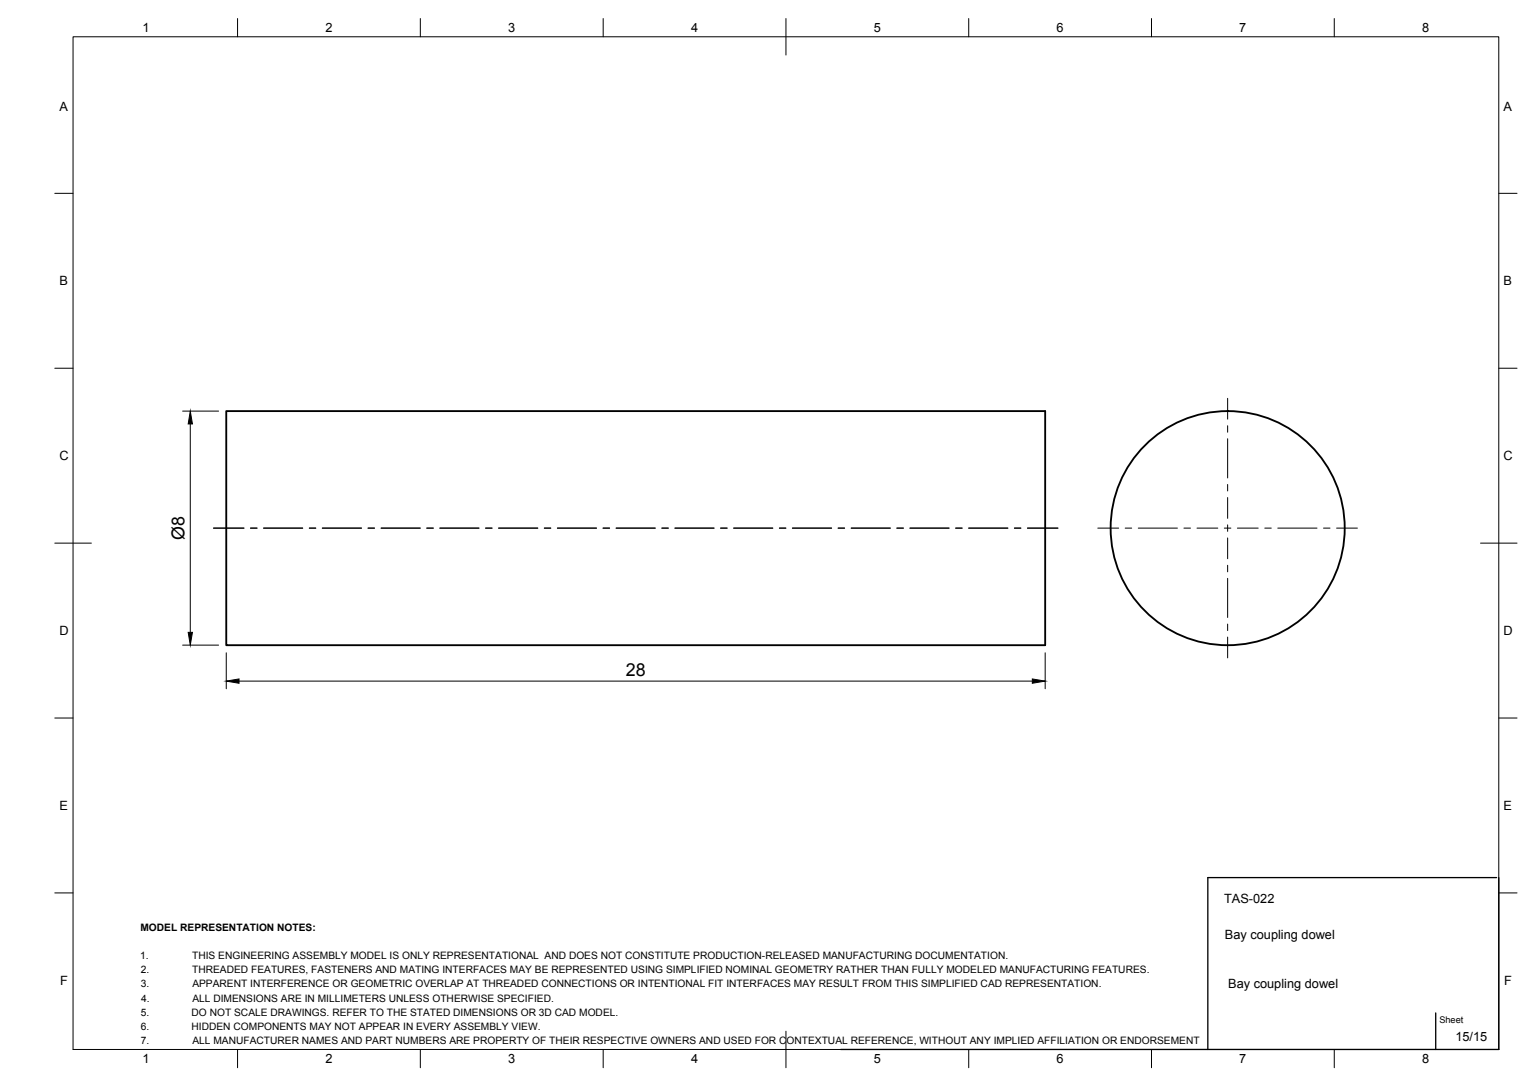
ISO-10303-21;
HEADER;
/* Generated by software containing ST-Developer
 * from STEP Tools, Inc. (www.steptools.com) 
 */

FILE_DESCRIPTION(
/* description */ (''),
/* implementation_level */ '2;1');

FILE_NAME(
/* name */ 'Bay coupling dowel.step',
/* time_stamp */ '2026-11-15T21:02:08-08:00',
/* author */ (''),
/* organization */ (''),
/* preprocessor_version */ 'ST-DEVELOPER v20.2',
/* originating_system */ 'Autodesk Translation Framework v15.17.0.0',
/* authorisation */ '');

FILE_SCHEMA (('AUTOMOTIVE_DESIGN { 1 0 10303 214 3 1 1 }'));
ENDSEC;

DATA;
#10=MECHANICAL_DESIGN_GEOMETRIC_PRESENTATION_REPRESENTATION('',(#616),#31566);
#488=CIRCLE('',#6246,0.4);
#489=CIRCLE('',#6247,0.4);
#571=CYLINDRICAL_SURFACE('',#6245,0.4);
#586=SHAPE_REPRESENTATION_RELATIONSHIP('SRR','None',#31650,#601);
#601=ADVANCED_BREP_SHAPE_REPRESENTATION('',(#631),#31565);
#616=STYLED_ITEM('',(#31725),#631);
#631=MANIFOLD_SOLID_BREP('Body1',#5729);
#898=FACE_OUTER_BOUND('',#1203,.T.);
#899=FACE_OUTER_BOUND('',#1204,.T.);
#900=FACE_OUTER_BOUND('',#1205,.T.);
#1203=EDGE_LOOP('',(#5257,#5258,#5259,#5260));
#1204=EDGE_LOOP('',(#5261));
#1205=EDGE_LOOP('',(#5262));
#1712=LINE('',#31497,#2219);
#2219=VECTOR('',#7490,0.4);
#2807=VERTEX_POINT('',#31494);
#2808=VERTEX_POINT('',#31496);
#3624=EDGE_CURVE('',#2807,#2807,#488,.T.);
#3625=EDGE_CURVE('',#2807,#2808,#1712,.T.);
#3626=EDGE_CURVE('',#2808,#2808,#489,.T.);
#5257=ORIENTED_EDGE('',*,*,#3624,.F.);
#5258=ORIENTED_EDGE('',*,*,#3625,.T.);
#5259=ORIENTED_EDGE('',*,*,#3626,.T.);
#5260=ORIENTED_EDGE('',*,*,#3625,.F.);
#5261=ORIENTED_EDGE('',*,*,#3624,.T.);
#5262=ORIENTED_EDGE('',*,*,#3626,.F.);
#5444=PLANE('',#6248);
#5445=PLANE('',#6249);
#5712=ADVANCED_FACE('',(#898),#571,.T.);
#5713=ADVANCED_FACE('',(#899),#5444,.T.);
#5714=ADVANCED_FACE('',(#900),#5445,.F.);
#5729=CLOSED_SHELL('',(#5712,#5713,#5714));
#6244=AXIS2_PLACEMENT_3D('',#31492,#7484,#7485);
#6245=AXIS2_PLACEMENT_3D('',#31493,#7486,#7487);
#6246=AXIS2_PLACEMENT_3D('',#31495,#7488,#7489);
#6247=AXIS2_PLACEMENT_3D('',#31498,#7491,#7492);
#6248=AXIS2_PLACEMENT_3D('',#31499,#7493,#7494);
#6249=AXIS2_PLACEMENT_3D('',#31500,#7495,#7496);
#7484=DIRECTION('axis',(0.,0.,1.));
#7485=DIRECTION('refdir',(1.,0.,0.));
#7486=DIRECTION('center_axis',(0.,0.,1.));
#7487=DIRECTION('ref_axis',(1.,0.,0.));
#7488=DIRECTION('center_axis',(0.,0.,1.));
#7489=DIRECTION('ref_axis',(1.,0.,0.));
#7490=DIRECTION('',(0.,0.,-1.));
#7491=DIRECTION('center_axis',(0.,0.,1.));
#7492=DIRECTION('ref_axis',(1.,0.,0.));
#7493=DIRECTION('center_axis',(0.,0.,1.));
#7494=DIRECTION('ref_axis',(1.,0.,0.));
#7495=DIRECTION('center_axis',(0.,0.,1.));
#7496=DIRECTION('ref_axis',(1.,0.,0.));
#31492=CARTESIAN_POINT('',(0.,0.,0.));
#31493=CARTESIAN_POINT('Origin',(0.,0.,0.));
#31494=CARTESIAN_POINT('',(-0.4,-4.89858719658941E-17,2.8));
#31495=CARTESIAN_POINT('Origin',(0.,0.,2.8));
#31496=CARTESIAN_POINT('',(-0.4,-4.89858719658941E-17,0.));
#31497=CARTESIAN_POINT('',(-0.4,-4.89858719658941E-17,0.));
#31498=CARTESIAN_POINT('Origin',(0.,0.,0.));
#31499=CARTESIAN_POINT('Origin',(0.,0.,2.8));
#31500=CARTESIAN_POINT('Origin',(0.,0.,0.));
#31548=UNCERTAINTY_MEASURE_WITH_UNIT(LENGTH_MEASURE(0.001),#31567,
'DISTANCE_ACCURACY_VALUE',
'Maximum model space distance between geometric entities at asserted c
onnectivities');
#31549=UNCERTAINTY_MEASURE_WITH_UNIT(LENGTH_MEASURE(0.001),#31567,
'DISTANCE_ACCURACY_VALUE',
'Maximum model space distance between geometric entities at asserted c
onnectivities');
#31565=(
GEOMETRIC_REPRESENTATION_CONTEXT(3)
GLOBAL_UNCERTAINTY_ASSIGNED_CONTEXT((#31548))
GLOBAL_UNIT_ASSIGNED_CONTEXT((#31567,#31569,#31570))
REPRESENTATION_CONTEXT('','3D')
);
#31566=(
GEOMETRIC_REPRESENTATION_CONTEXT(3)
GLOBAL_UNCERTAINTY_ASSIGNED_CONTEXT((#31549))
GLOBAL_UNIT_ASSIGNED_CONTEXT((#31567,#31569,#31570))
REPRESENTATION_CONTEXT('','3D')
);
#31567=(
LENGTH_UNIT()
NAMED_UNIT(*)
SI_UNIT(.CENTI.,.METRE.)
);
#31569=(
NAMED_UNIT(*)
PLANE_ANGLE_UNIT()
SI_UNIT($,.RADIAN.)
);
#31570=(
NAMED_UNIT(*)
SI_UNIT($,.STERADIAN.)
SOLID_ANGLE_UNIT()
);
#31586=SHAPE_DEFINITION_REPRESENTATION(#31602,#31650);
#31602=PRODUCT_DEFINITION_SHAPE('',$,#31667);
#31650=SHAPE_REPRESENTATION('',(#6244),#31565);
#31651=PRODUCT_DEFINITION_CONTEXT('part definition',#31701,'design');
#31667=PRODUCT_DEFINITION('Bay coupling dowel','Bay coupling dowel',#31683,
#31651);
#31683=PRODUCT_DEFINITION_FORMATION('',$,#31718);
#31701=APPLICATION_CONTEXT(
'Core Data for Automotive Mechanical Design Process');
#31702=PRODUCT_CONTEXT('part definition',#31701,'mechanical');
#31718=PRODUCT('Bay coupling dowel','Bay coupling dowel',$,(#31702));
#31725=PRESENTATION_STYLE_ASSIGNMENT((#31732));
#31732=SURFACE_STYLE_USAGE(.BOTH.,#31739);
#31739=SURFACE_SIDE_STYLE('',(#31746));
#31746=SURFACE_STYLE_FILL_AREA(#31753);
#31753=FILL_AREA_STYLE('Opaque(112,122,133)',(#31760));
#31760=FILL_AREA_STYLE_COLOUR('Opaque(112,122,133)',#31767);
#31767=COLOUR_RGB('Opaque(112,122,133)',0.43921568627451,0.47843137254902,
0.52156862745098);
ENDSEC;
END-ISO-10303-21;
